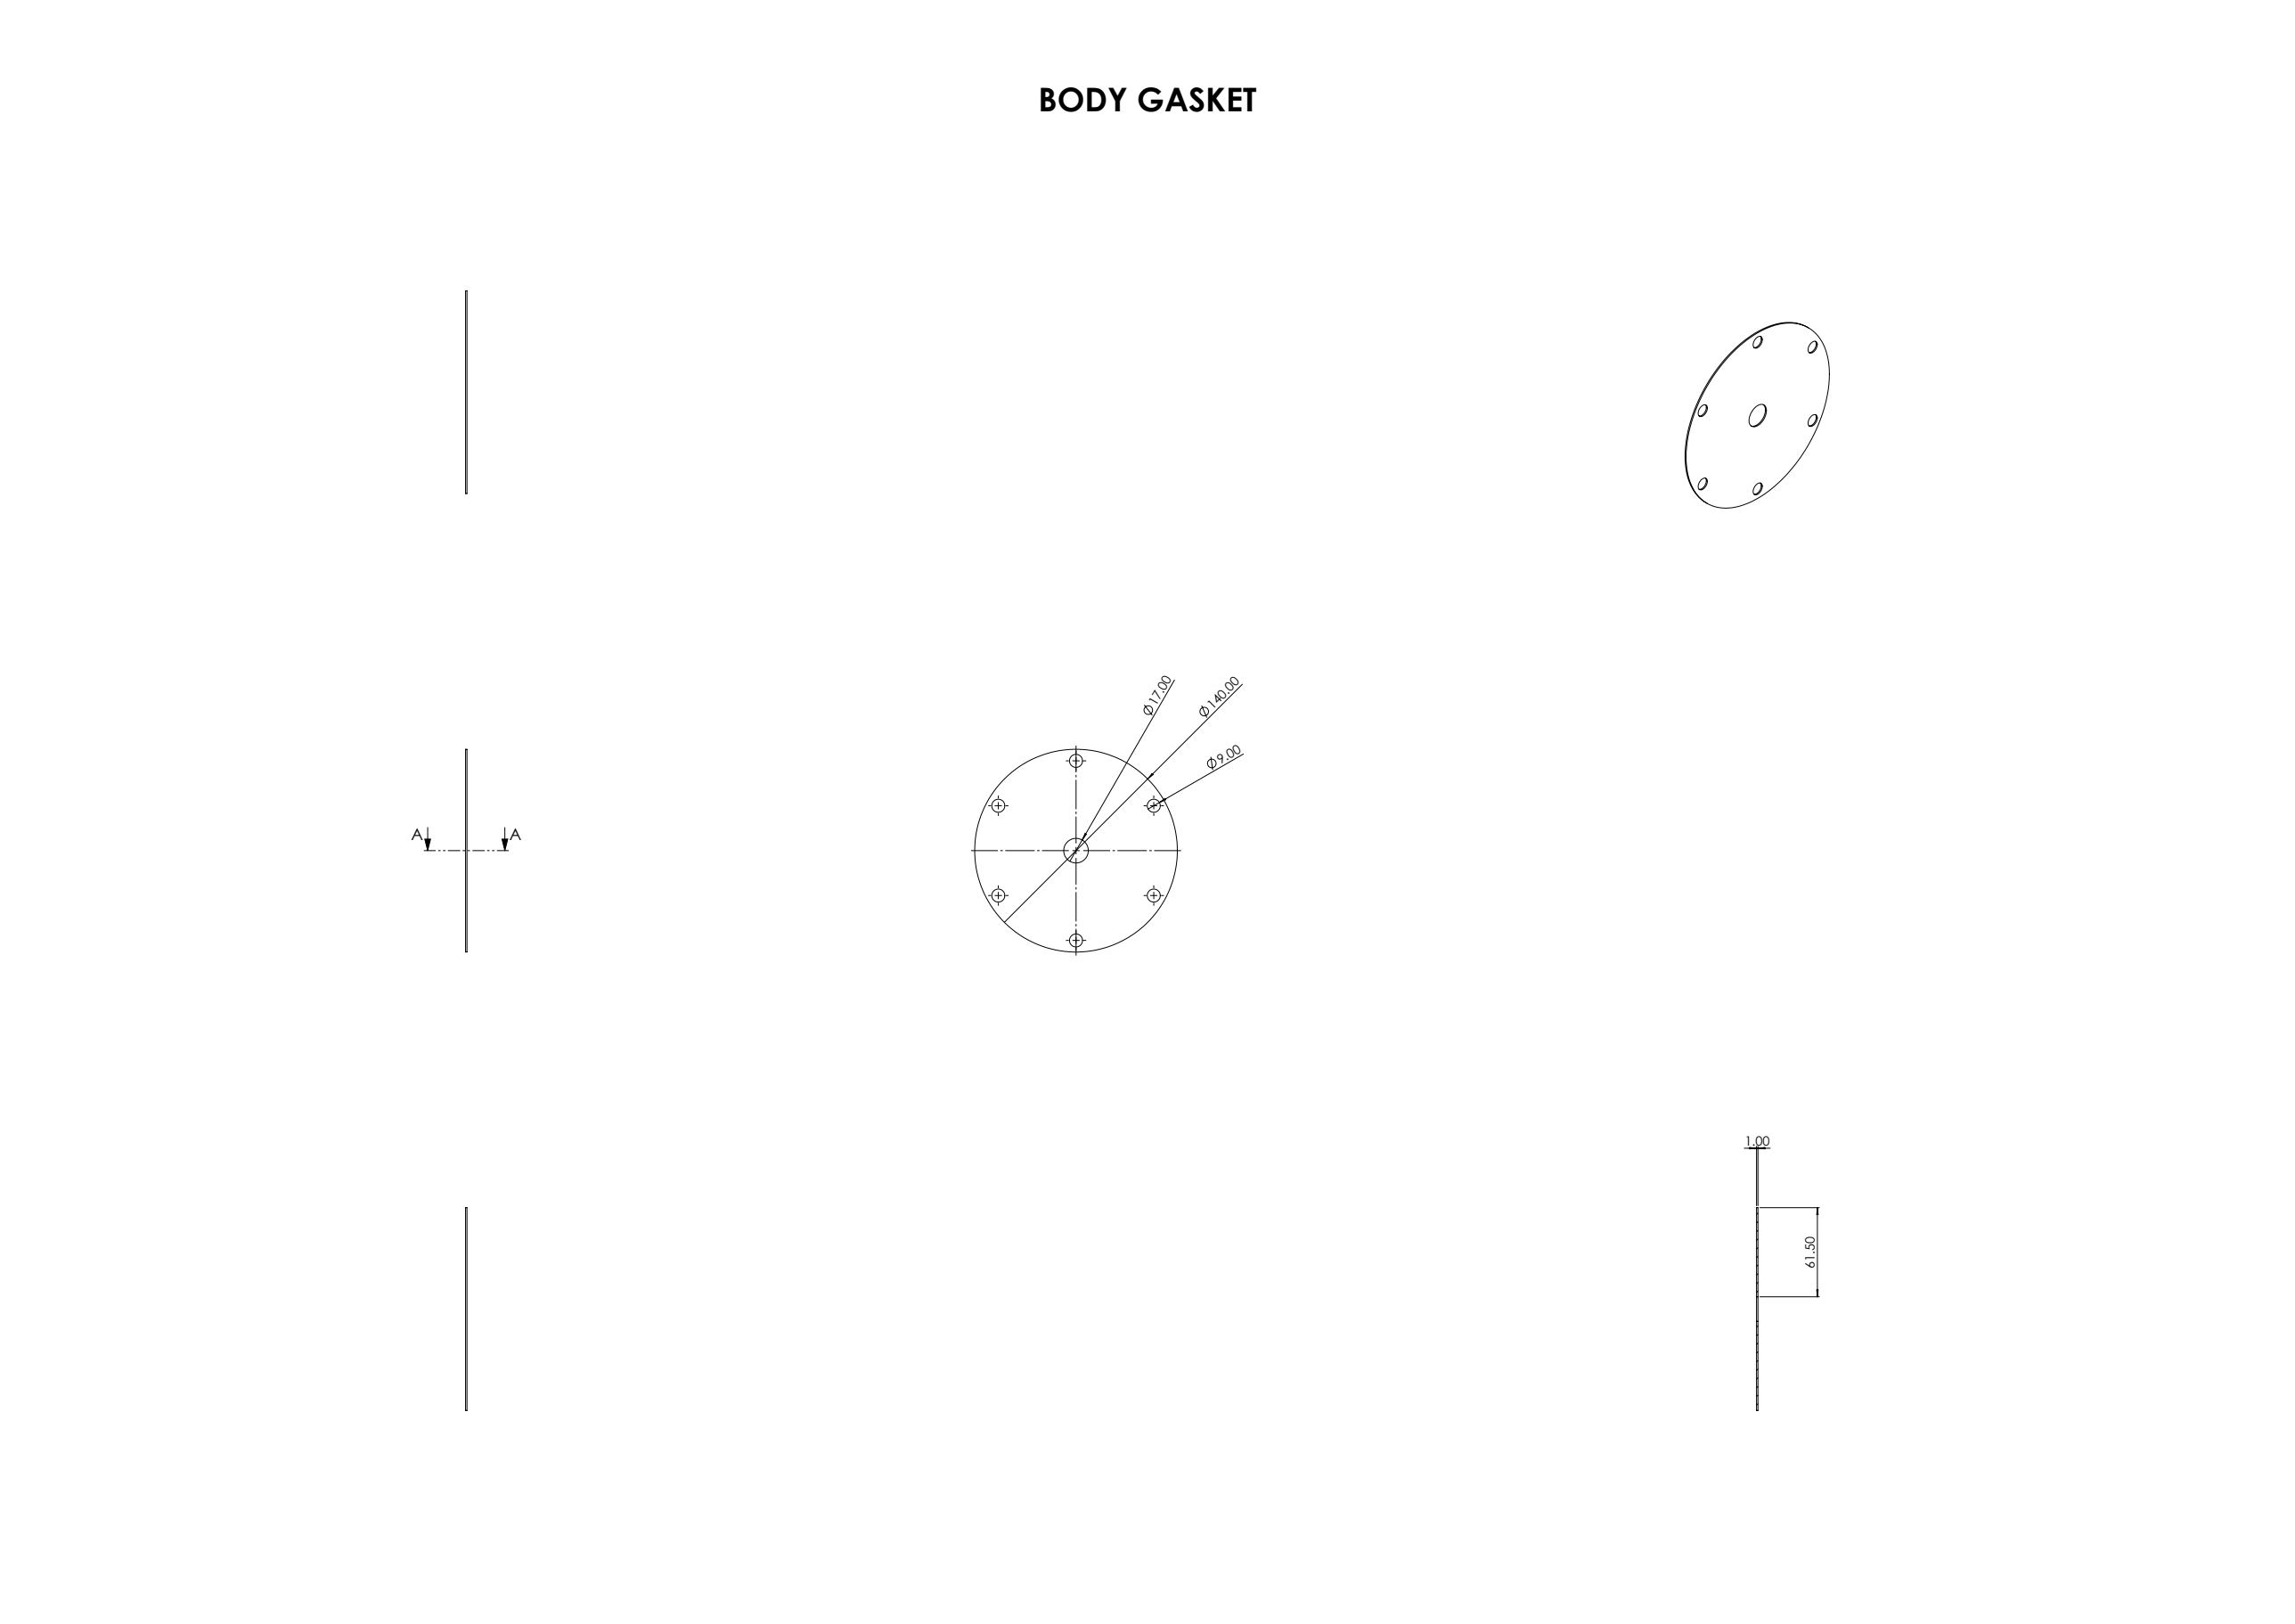
ISO-10303-21;
HEADER;
/* Generated by software containing ST-Developer
 * from STEP Tools, Inc. (www.steptools.com) 
 */

FILE_DESCRIPTION(
/* description */ (''),
/* implementation_level */ '2;1');

FILE_NAME(
/* name */ '04_Body_Gasket.step',
/* time_stamp */ '2026-10-26T06:13:19-07:00',
/* author */ (''),
/* organization */ (''),
/* preprocessor_version */ 'ST-DEVELOPER v20.2',
/* originating_system */ 'Autodesk Translation Framework v15.15.0.0',
/* authorisation */ '');

FILE_SCHEMA (('AUTOMOTIVE_DESIGN { 1 0 10303 214 3 1 1 }','TECHNICAL_DATA_PACKAGING'));
ENDSEC;

DATA;
#10=MECHANICAL_DESIGN_GEOMETRIC_PRESENTATION_REPRESENTATION('',(#300),#56639);
#260=SHAPE_REPRESENTATION_RELATIONSHIP('SRR','None',#56748,#280);
#280=ADVANCED_BREP_SHAPE_REPRESENTATION('',(#320),#56622);
#300=STYLED_ITEM('',(#56894),#320);
#320=MANIFOLD_SOLID_BREP('Body1',#16952);
#476=FACE_BOUND('',#3034,.T.);
#477=FACE_BOUND('',#3035,.T.);
#478=FACE_BOUND('',#3036,.T.);
#479=FACE_BOUND('',#3037,.T.);
#480=FACE_BOUND('',#3038,.T.);
#481=FACE_BOUND('',#3039,.T.);
#482=FACE_BOUND('',#3040,.T.);
#483=FACE_BOUND('',#3043,.T.);
#484=FACE_BOUND('',#3044,.T.);
#485=FACE_BOUND('',#3045,.T.);
#486=FACE_BOUND('',#3046,.T.);
#487=FACE_BOUND('',#3047,.T.);
#488=FACE_BOUND('',#3048,.T.);
#489=FACE_BOUND('',#3049,.T.);
#872=CIRCLE('',#17590,4.5);
#873=CIRCLE('',#17591,4.5);
#874=CIRCLE('',#17593,4.5);
#875=CIRCLE('',#17594,4.5);
#876=CIRCLE('',#17596,4.5);
#877=CIRCLE('',#17597,4.5);
#878=CIRCLE('',#17599,4.5);
#879=CIRCLE('',#17600,4.5);
#880=CIRCLE('',#17602,4.5);
#881=CIRCLE('',#17603,4.5);
#882=CIRCLE('',#17605,4.5);
#883=CIRCLE('',#17606,4.5);
#884=CIRCLE('',#17608,8.5);
#885=CIRCLE('',#17609,8.5);
#886=CIRCLE('',#17611,70.);
#887=CIRCLE('',#17613,70.);
#1301=CYLINDRICAL_SURFACE('',#17589,4.5);
#1302=CYLINDRICAL_SURFACE('',#17592,4.5);
#1303=CYLINDRICAL_SURFACE('',#17595,4.5);
#1304=CYLINDRICAL_SURFACE('',#17598,4.5);
#1305=CYLINDRICAL_SURFACE('',#17601,4.5);
#1306=CYLINDRICAL_SURFACE('',#17604,4.5);
#1307=CYLINDRICAL_SURFACE('',#17607,8.5);
#1308=CYLINDRICAL_SURFACE('',#17612,70.);
#1991=FACE_OUTER_BOUND('',#3026,.T.);
#1992=FACE_OUTER_BOUND('',#3027,.T.);
#1993=FACE_OUTER_BOUND('',#3028,.T.);
#1994=FACE_OUTER_BOUND('',#3029,.T.);
#1995=FACE_OUTER_BOUND('',#3030,.T.);
#1996=FACE_OUTER_BOUND('',#3031,.T.);
#1997=FACE_OUTER_BOUND('',#3032,.T.);
#1998=FACE_OUTER_BOUND('',#3033,.T.);
#1999=FACE_OUTER_BOUND('',#3041,.T.);
#2000=FACE_OUTER_BOUND('',#3042,.T.);
#3026=EDGE_LOOP('',(#11684,#11685,#11686,#11687));
#3027=EDGE_LOOP('',(#11688,#11689,#11690,#11691));
#3028=EDGE_LOOP('',(#11692,#11693,#11694,#11695));
#3029=EDGE_LOOP('',(#11696,#11697,#11698,#11699));
#3030=EDGE_LOOP('',(#11700,#11701,#11702,#11703));
#3031=EDGE_LOOP('',(#11704,#11705,#11706,#11707));
#3032=EDGE_LOOP('',(#11708,#11709,#11710,#11711));
#3033=EDGE_LOOP('',(#11712));
#3034=EDGE_LOOP('',(#11713));
#3035=EDGE_LOOP('',(#11714));
#3036=EDGE_LOOP('',(#11715));
#3037=EDGE_LOOP('',(#11716));
#3038=EDGE_LOOP('',(#11717));
#3039=EDGE_LOOP('',(#11718));
#3040=EDGE_LOOP('',(#11719));
#3041=EDGE_LOOP('',(#11720,#11721,#11722,#11723));
#3042=EDGE_LOOP('',(#11724));
#3043=EDGE_LOOP('',(#11725));
#3044=EDGE_LOOP('',(#11726));
#3045=EDGE_LOOP('',(#11727));
#3046=EDGE_LOOP('',(#11728));
#3047=EDGE_LOOP('',(#11729));
#3048=EDGE_LOOP('',(#11730));
#3049=EDGE_LOOP('',(#11731));
#4075=LINE('',#24948,#5029);
#4076=LINE('',#24954,#5030);
#4077=LINE('',#24960,#5031);
#4078=LINE('',#24966,#5032);
#4079=LINE('',#24972,#5033);
#4080=LINE('',#24978,#5034);
#4081=LINE('',#24984,#5035);
#4082=LINE('',#24992,#5036);
#5029=VECTOR('',#19765,4.5);
#5030=VECTOR('',#19772,4.5);
#5031=VECTOR('',#19779,4.5);
#5032=VECTOR('',#19786,4.5);
#5033=VECTOR('',#19793,4.5);
#5034=VECTOR('',#19800,4.5);
#5035=VECTOR('',#19807,8.5);
#5036=VECTOR('',#19818,70.);
#7003=VERTEX_POINT('',#24945);
#7004=VERTEX_POINT('',#24947);
#7005=VERTEX_POINT('',#24951);
#7006=VERTEX_POINT('',#24953);
#7007=VERTEX_POINT('',#24957);
#7008=VERTEX_POINT('',#24959);
#7009=VERTEX_POINT('',#24963);
#7010=VERTEX_POINT('',#24965);
#7011=VERTEX_POINT('',#24969);
#7012=VERTEX_POINT('',#24971);
#7013=VERTEX_POINT('',#24975);
#7014=VERTEX_POINT('',#24977);
#7015=VERTEX_POINT('',#24981);
#7016=VERTEX_POINT('',#24983);
#7017=VERTEX_POINT('',#24987);
#7018=VERTEX_POINT('',#24990);
#8749=EDGE_CURVE('',#7003,#7003,#872,.T.);
#8750=EDGE_CURVE('',#7003,#7004,#4075,.T.);
#8751=EDGE_CURVE('',#7004,#7004,#873,.T.);
#8752=EDGE_CURVE('',#7005,#7005,#874,.T.);
#8753=EDGE_CURVE('',#7005,#7006,#4076,.T.);
#8754=EDGE_CURVE('',#7006,#7006,#875,.T.);
#8755=EDGE_CURVE('',#7007,#7007,#876,.T.);
#8756=EDGE_CURVE('',#7007,#7008,#4077,.T.);
#8757=EDGE_CURVE('',#7008,#7008,#877,.T.);
#8758=EDGE_CURVE('',#7009,#7009,#878,.T.);
#8759=EDGE_CURVE('',#7009,#7010,#4078,.T.);
#8760=EDGE_CURVE('',#7010,#7010,#879,.T.);
#8761=EDGE_CURVE('',#7011,#7011,#880,.T.);
#8762=EDGE_CURVE('',#7011,#7012,#4079,.T.);
#8763=EDGE_CURVE('',#7012,#7012,#881,.T.);
#8764=EDGE_CURVE('',#7013,#7013,#882,.T.);
#8765=EDGE_CURVE('',#7013,#7014,#4080,.T.);
#8766=EDGE_CURVE('',#7014,#7014,#883,.T.);
#8767=EDGE_CURVE('',#7015,#7015,#884,.T.);
#8768=EDGE_CURVE('',#7015,#7016,#4081,.T.);
#8769=EDGE_CURVE('',#7016,#7016,#885,.T.);
#8770=EDGE_CURVE('',#7017,#7017,#886,.T.);
#8771=EDGE_CURVE('',#7018,#7018,#887,.T.);
#8772=EDGE_CURVE('',#7018,#7017,#4082,.T.);
#11684=ORIENTED_EDGE('',*,*,#8749,.F.);
#11685=ORIENTED_EDGE('',*,*,#8750,.T.);
#11686=ORIENTED_EDGE('',*,*,#8751,.F.);
#11687=ORIENTED_EDGE('',*,*,#8750,.F.);
#11688=ORIENTED_EDGE('',*,*,#8752,.F.);
#11689=ORIENTED_EDGE('',*,*,#8753,.T.);
#11690=ORIENTED_EDGE('',*,*,#8754,.F.);
#11691=ORIENTED_EDGE('',*,*,#8753,.F.);
#11692=ORIENTED_EDGE('',*,*,#8755,.F.);
#11693=ORIENTED_EDGE('',*,*,#8756,.T.);
#11694=ORIENTED_EDGE('',*,*,#8757,.F.);
#11695=ORIENTED_EDGE('',*,*,#8756,.F.);
#11696=ORIENTED_EDGE('',*,*,#8758,.F.);
#11697=ORIENTED_EDGE('',*,*,#8759,.T.);
#11698=ORIENTED_EDGE('',*,*,#8760,.F.);
#11699=ORIENTED_EDGE('',*,*,#8759,.F.);
#11700=ORIENTED_EDGE('',*,*,#8761,.F.);
#11701=ORIENTED_EDGE('',*,*,#8762,.T.);
#11702=ORIENTED_EDGE('',*,*,#8763,.F.);
#11703=ORIENTED_EDGE('',*,*,#8762,.F.);
#11704=ORIENTED_EDGE('',*,*,#8764,.F.);
#11705=ORIENTED_EDGE('',*,*,#8765,.T.);
#11706=ORIENTED_EDGE('',*,*,#8766,.F.);
#11707=ORIENTED_EDGE('',*,*,#8765,.F.);
#11708=ORIENTED_EDGE('',*,*,#8767,.T.);
#11709=ORIENTED_EDGE('',*,*,#8768,.T.);
#11710=ORIENTED_EDGE('',*,*,#8769,.F.);
#11711=ORIENTED_EDGE('',*,*,#8768,.F.);
#11712=ORIENTED_EDGE('',*,*,#8770,.F.);
#11713=ORIENTED_EDGE('',*,*,#8769,.T.);
#11714=ORIENTED_EDGE('',*,*,#8764,.T.);
#11715=ORIENTED_EDGE('',*,*,#8761,.T.);
#11716=ORIENTED_EDGE('',*,*,#8758,.T.);
#11717=ORIENTED_EDGE('',*,*,#8755,.T.);
#11718=ORIENTED_EDGE('',*,*,#8752,.T.);
#11719=ORIENTED_EDGE('',*,*,#8749,.T.);
#11720=ORIENTED_EDGE('',*,*,#8771,.F.);
#11721=ORIENTED_EDGE('',*,*,#8772,.T.);
#11722=ORIENTED_EDGE('',*,*,#8770,.T.);
#11723=ORIENTED_EDGE('',*,*,#8772,.F.);
#11724=ORIENTED_EDGE('',*,*,#8771,.T.);
#11725=ORIENTED_EDGE('',*,*,#8767,.F.);
#11726=ORIENTED_EDGE('',*,*,#8766,.T.);
#11727=ORIENTED_EDGE('',*,*,#8763,.T.);
#11728=ORIENTED_EDGE('',*,*,#8760,.T.);
#11729=ORIENTED_EDGE('',*,*,#8757,.T.);
#11730=ORIENTED_EDGE('',*,*,#8754,.T.);
#11731=ORIENTED_EDGE('',*,*,#8751,.T.);
#15773=PLANE('',#17610);
#15774=PLANE('',#17614);
#16162=ADVANCED_FACE('',(#1991),#1301,.F.);
#16163=ADVANCED_FACE('',(#1992),#1302,.F.);
#16164=ADVANCED_FACE('',(#1993),#1303,.F.);
#16165=ADVANCED_FACE('',(#1994),#1304,.F.);
#16166=ADVANCED_FACE('',(#1995),#1305,.F.);
#16167=ADVANCED_FACE('',(#1996),#1306,.F.);
#16168=ADVANCED_FACE('',(#1997),#1307,.F.);
#16169=ADVANCED_FACE('',(#1998,#476,#477,#478,#479,#480,#481,#482),#15773,
 .T.);
#16170=ADVANCED_FACE('',(#1999),#1308,.T.);
#16171=ADVANCED_FACE('',(#2000,#483,#484,#485,#486,#487,#488,#489),#15774,
 .T.);
#16952=CLOSED_SHELL('',(#16162,#16163,#16164,#16165,#16166,#16167,#16168,
#16169,#16170,#16171));
#17588=AXIS2_PLACEMENT_3D('',#24943,#19759,#19760);
#17589=AXIS2_PLACEMENT_3D('',#24944,#19761,#19762);
#17590=AXIS2_PLACEMENT_3D('',#24946,#19763,#19764);
#17591=AXIS2_PLACEMENT_3D('',#24949,#19766,#19767);
#17592=AXIS2_PLACEMENT_3D('',#24950,#19768,#19769);
#17593=AXIS2_PLACEMENT_3D('',#24952,#19770,#19771);
#17594=AXIS2_PLACEMENT_3D('',#24955,#19773,#19774);
#17595=AXIS2_PLACEMENT_3D('',#24956,#19775,#19776);
#17596=AXIS2_PLACEMENT_3D('',#24958,#19777,#19778);
#17597=AXIS2_PLACEMENT_3D('',#24961,#19780,#19781);
#17598=AXIS2_PLACEMENT_3D('',#24962,#19782,#19783);
#17599=AXIS2_PLACEMENT_3D('',#24964,#19784,#19785);
#17600=AXIS2_PLACEMENT_3D('',#24967,#19787,#19788);
#17601=AXIS2_PLACEMENT_3D('',#24968,#19789,#19790);
#17602=AXIS2_PLACEMENT_3D('',#24970,#19791,#19792);
#17603=AXIS2_PLACEMENT_3D('',#24973,#19794,#19795);
#17604=AXIS2_PLACEMENT_3D('',#24974,#19796,#19797);
#17605=AXIS2_PLACEMENT_3D('',#24976,#19798,#19799);
#17606=AXIS2_PLACEMENT_3D('',#24979,#19801,#19802);
#17607=AXIS2_PLACEMENT_3D('',#24980,#19803,#19804);
#17608=AXIS2_PLACEMENT_3D('',#24982,#19805,#19806);
#17609=AXIS2_PLACEMENT_3D('',#24985,#19808,#19809);
#17610=AXIS2_PLACEMENT_3D('',#24986,#19810,#19811);
#17611=AXIS2_PLACEMENT_3D('',#24988,#19812,#19813);
#17612=AXIS2_PLACEMENT_3D('',#24989,#19814,#19815);
#17613=AXIS2_PLACEMENT_3D('',#24991,#19816,#19817);
#17614=AXIS2_PLACEMENT_3D('',#24993,#19819,#19820);
#19759=DIRECTION('axis',(0.,0.,1.));
#19760=DIRECTION('refdir',(1.,0.,0.));
#19761=DIRECTION('center_axis',(1.,0.,0.));
#19762=DIRECTION('ref_axis',(0.,0.,-1.));
#19763=DIRECTION('center_axis',(1.,0.,0.));
#19764=DIRECTION('ref_axis',(0.,0.,-1.));
#19765=DIRECTION('',(1.,0.,0.));
#19766=DIRECTION('center_axis',(-1.,0.,0.));
#19767=DIRECTION('ref_axis',(0.,0.,-1.));
#19768=DIRECTION('center_axis',(1.,0.,0.));
#19769=DIRECTION('ref_axis',(0.,0.,-1.));
#19770=DIRECTION('center_axis',(1.,0.,0.));
#19771=DIRECTION('ref_axis',(0.,0.,-1.));
#19772=DIRECTION('',(1.,0.,0.));
#19773=DIRECTION('center_axis',(-1.,0.,0.));
#19774=DIRECTION('ref_axis',(0.,0.,-1.));
#19775=DIRECTION('center_axis',(1.,0.,0.));
#19776=DIRECTION('ref_axis',(0.,0.,-1.));
#19777=DIRECTION('center_axis',(1.,0.,0.));
#19778=DIRECTION('ref_axis',(0.,0.,-1.));
#19779=DIRECTION('',(1.,0.,0.));
#19780=DIRECTION('center_axis',(-1.,0.,0.));
#19781=DIRECTION('ref_axis',(0.,0.,-1.));
#19782=DIRECTION('center_axis',(1.,0.,0.));
#19783=DIRECTION('ref_axis',(0.,0.,-1.));
#19784=DIRECTION('center_axis',(1.,0.,0.));
#19785=DIRECTION('ref_axis',(0.,0.,-1.));
#19786=DIRECTION('',(1.,0.,0.));
#19787=DIRECTION('center_axis',(-1.,0.,0.));
#19788=DIRECTION('ref_axis',(0.,0.,-1.));
#19789=DIRECTION('center_axis',(1.,0.,0.));
#19790=DIRECTION('ref_axis',(0.,0.,-1.));
#19791=DIRECTION('center_axis',(1.,0.,0.));
#19792=DIRECTION('ref_axis',(0.,0.,-1.));
#19793=DIRECTION('',(1.,0.,0.));
#19794=DIRECTION('center_axis',(-1.,0.,0.));
#19795=DIRECTION('ref_axis',(0.,0.,-1.));
#19796=DIRECTION('center_axis',(1.,0.,0.));
#19797=DIRECTION('ref_axis',(0.,0.,-1.));
#19798=DIRECTION('center_axis',(1.,0.,0.));
#19799=DIRECTION('ref_axis',(0.,0.,-1.));
#19800=DIRECTION('',(1.,0.,0.));
#19801=DIRECTION('center_axis',(-1.,0.,0.));
#19802=DIRECTION('ref_axis',(0.,0.,-1.));
#19803=DIRECTION('center_axis',(1.,0.,0.));
#19804=DIRECTION('ref_axis',(0.,1.,0.));
#19805=DIRECTION('center_axis',(1.,0.,0.));
#19806=DIRECTION('ref_axis',(0.,0.,-1.));
#19807=DIRECTION('',(-1.,0.,0.));
#19808=DIRECTION('center_axis',(1.,0.,0.));
#19809=DIRECTION('ref_axis',(0.,0.,-1.));
#19810=DIRECTION('center_axis',(-1.,0.,0.));
#19811=DIRECTION('ref_axis',(0.,0.,1.));
#19812=DIRECTION('center_axis',(1.,0.,0.));
#19813=DIRECTION('ref_axis',(0.,0.,-1.));
#19814=DIRECTION('center_axis',(1.,0.,0.));
#19815=DIRECTION('ref_axis',(0.,1.,0.));
#19816=DIRECTION('center_axis',(1.,0.,0.));
#19817=DIRECTION('ref_axis',(0.,0.,-1.));
#19818=DIRECTION('',(-1.,0.,0.));
#19819=DIRECTION('center_axis',(1.,0.,0.));
#19820=DIRECTION('ref_axis',(0.,0.,-1.));
#24943=CARTESIAN_POINT('',(0.,0.,0.));
#24944=CARTESIAN_POINT('Origin',(-0.6,-31.,-53.6935750346352));
#24945=CARTESIAN_POINT('',(-0.5,-31.,-49.1935750346352));
#24946=CARTESIAN_POINT('Origin',(-0.5,-31.,-53.6935750346352));
#24947=CARTESIAN_POINT('',(0.5,-31.,-49.1935750346352));
#24948=CARTESIAN_POINT('',(-0.6,-31.,-49.1935750346352));
#24949=CARTESIAN_POINT('Origin',(0.5,-31.,-53.6935750346352));
#24950=CARTESIAN_POINT('Origin',(-0.6,62.,0.));
#24951=CARTESIAN_POINT('',(-0.5,62.,4.5));
#24952=CARTESIAN_POINT('Origin',(-0.5,62.,0.));
#24953=CARTESIAN_POINT('',(0.5,62.,4.5));
#24954=CARTESIAN_POINT('',(-0.6,62.,4.5));
#24955=CARTESIAN_POINT('Origin',(0.5,62.,0.));
#24956=CARTESIAN_POINT('Origin',(-0.6,31.,53.6935750346352));
#24957=CARTESIAN_POINT('',(-0.5,31.,58.1935750346352));
#24958=CARTESIAN_POINT('Origin',(-0.5,31.,53.6935750346352));
#24959=CARTESIAN_POINT('',(0.5,31.,58.1935750346352));
#24960=CARTESIAN_POINT('',(-0.6,31.,58.1935750346352));
#24961=CARTESIAN_POINT('Origin',(0.5,31.,53.6935750346352));
#24962=CARTESIAN_POINT('Origin',(-0.6,-31.,53.6935750346352));
#24963=CARTESIAN_POINT('',(-0.5,-31.,58.1935750346352));
#24964=CARTESIAN_POINT('Origin',(-0.5,-31.,53.6935750346352));
#24965=CARTESIAN_POINT('',(0.5,-31.,58.1935750346352));
#24966=CARTESIAN_POINT('',(-0.6,-31.,58.1935750346352));
#24967=CARTESIAN_POINT('Origin',(0.5,-31.,53.6935750346352));
#24968=CARTESIAN_POINT('Origin',(-0.6,-62.,7.59281015471359E-15));
#24969=CARTESIAN_POINT('',(-0.5,-62.,4.50000000000001));
#24970=CARTESIAN_POINT('Origin',(-0.5,-62.,7.59281015471359E-15));
#24971=CARTESIAN_POINT('',(0.5,-62.,4.50000000000001));
#24972=CARTESIAN_POINT('',(-0.6,-62.,4.50000000000001));
#24973=CARTESIAN_POINT('Origin',(0.5,-62.,7.59281015471359E-15));
#24974=CARTESIAN_POINT('Origin',(-0.6,31.,-53.6935750346352));
#24975=CARTESIAN_POINT('',(-0.5,31.,-49.1935750346352));
#24976=CARTESIAN_POINT('Origin',(-0.5,31.,-53.6935750346352));
#24977=CARTESIAN_POINT('',(0.5,31.,-49.1935750346352));
#24978=CARTESIAN_POINT('',(-0.6,31.,-49.1935750346352));
#24979=CARTESIAN_POINT('Origin',(0.5,31.,-53.6935750346352));
#24980=CARTESIAN_POINT('Origin',(0.,0.,0.));
#24981=CARTESIAN_POINT('',(0.5,-8.5,-1.04094977927525E-15));
#24982=CARTESIAN_POINT('Origin',(0.5,0.,0.));
#24983=CARTESIAN_POINT('',(-0.5,-8.5,-1.04094977927525E-15));
#24984=CARTESIAN_POINT('',(0.,-8.5,-1.04094977927525E-15));
#24985=CARTESIAN_POINT('Origin',(-0.5,0.,0.));
#24986=CARTESIAN_POINT('Origin',(-0.5,70.,0.));
#24987=CARTESIAN_POINT('',(-0.5,-70.,-8.57252759403147E-15));
#24988=CARTESIAN_POINT('Origin',(-0.5,0.,0.));
#24989=CARTESIAN_POINT('Origin',(0.,0.,0.));
#24990=CARTESIAN_POINT('',(0.5,-70.,-8.57252759403147E-15));
#24991=CARTESIAN_POINT('Origin',(0.5,0.,0.));
#24992=CARTESIAN_POINT('',(0.,-70.,-8.57252759403147E-15));
#24993=CARTESIAN_POINT('Origin',(0.5,8.5,0.));
#56600=UNCERTAINTY_MEASURE_WITH_UNIT(LENGTH_MEASURE(0.01),#56640,
'DISTANCE_ACCURACY_VALUE',
'Maximum model space distance between geometric entities at asserted c
onnectivities');
#56617=UNCERTAINTY_MEASURE_WITH_UNIT(LENGTH_MEASURE(0.01),#56640,
'DISTANCE_ACCURACY_VALUE',
'Maximum model space distance between geometric entities at asserted c
onnectivities');
#56622=(
GEOMETRIC_REPRESENTATION_CONTEXT(3)
GLOBAL_UNCERTAINTY_ASSIGNED_CONTEXT((#56600))
GLOBAL_UNIT_ASSIGNED_CONTEXT((#56640,#56642,#56643))
REPRESENTATION_CONTEXT('','3D')
);
#56639=(
GEOMETRIC_REPRESENTATION_CONTEXT(3)
GLOBAL_UNCERTAINTY_ASSIGNED_CONTEXT((#56617))
GLOBAL_UNIT_ASSIGNED_CONTEXT((#56640,#56642,#56643))
REPRESENTATION_CONTEXT('','3D')
);
#56640=(
LENGTH_UNIT()
NAMED_UNIT(*)
SI_UNIT(.MILLI.,.METRE.)
);
#56642=(
NAMED_UNIT(*)
PLANE_ANGLE_UNIT()
SI_UNIT($,.RADIAN.)
);
#56643=(
NAMED_UNIT(*)
SI_UNIT($,.STERADIAN.)
SOLID_ANGLE_UNIT()
);
#56648=SHAPE_DEFINITION_REPRESENTATION(#56669,#56748);
#56669=PRODUCT_DEFINITION_SHAPE('',$,#56770);
#56748=SHAPE_REPRESENTATION('',(#17588),#56622);
#56765=PRODUCT_DEFINITION_CONTEXT('part definition',#56830,'design');
#56770=PRODUCT_DEFINITION('2026-10-26-00-02-40-929','04_Body_Gasket',#56791,
#56765);
#56791=PRODUCT_DEFINITION_FORMATION('',$,#56836);
#56830=APPLICATION_CONTEXT(
'Core Data for Automotive Mechanical Design Process');
#56831=PRODUCT_CONTEXT('part definition',#56830,'mechanical');
#56836=PRODUCT('2026-10-26-00-02-40-929','04_Body_Gasket',$,(#56831));
#56888=COLOUR_RGB('Dark Blue',0.08,0.2,0.34);
#56889=FILL_AREA_STYLE_COLOUR('',#56888);
#56890=FILL_AREA_STYLE('',(#56889));
#56891=SURFACE_STYLE_FILL_AREA(#56890);
#56892=SURFACE_SIDE_STYLE('',(#56891));
#56893=SURFACE_STYLE_USAGE(.BOTH.,#56892);
#56894=PRESENTATION_STYLE_ASSIGNMENT((#56893));
ENDSEC;
END-ISO-10303-21;
